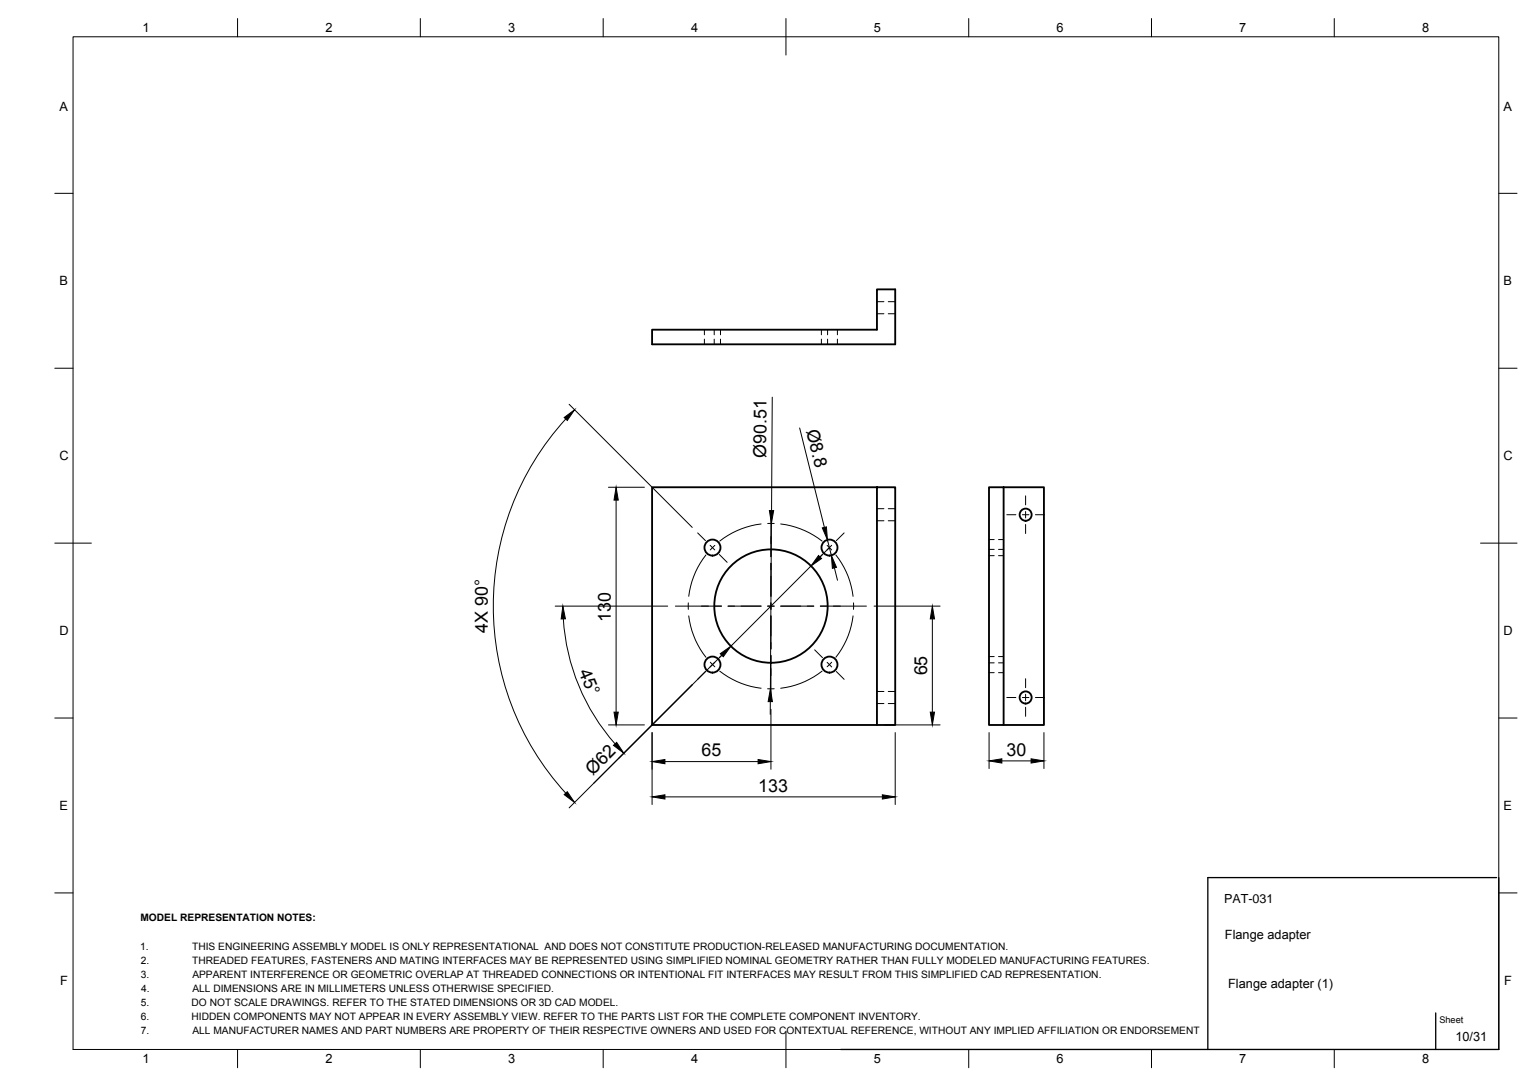
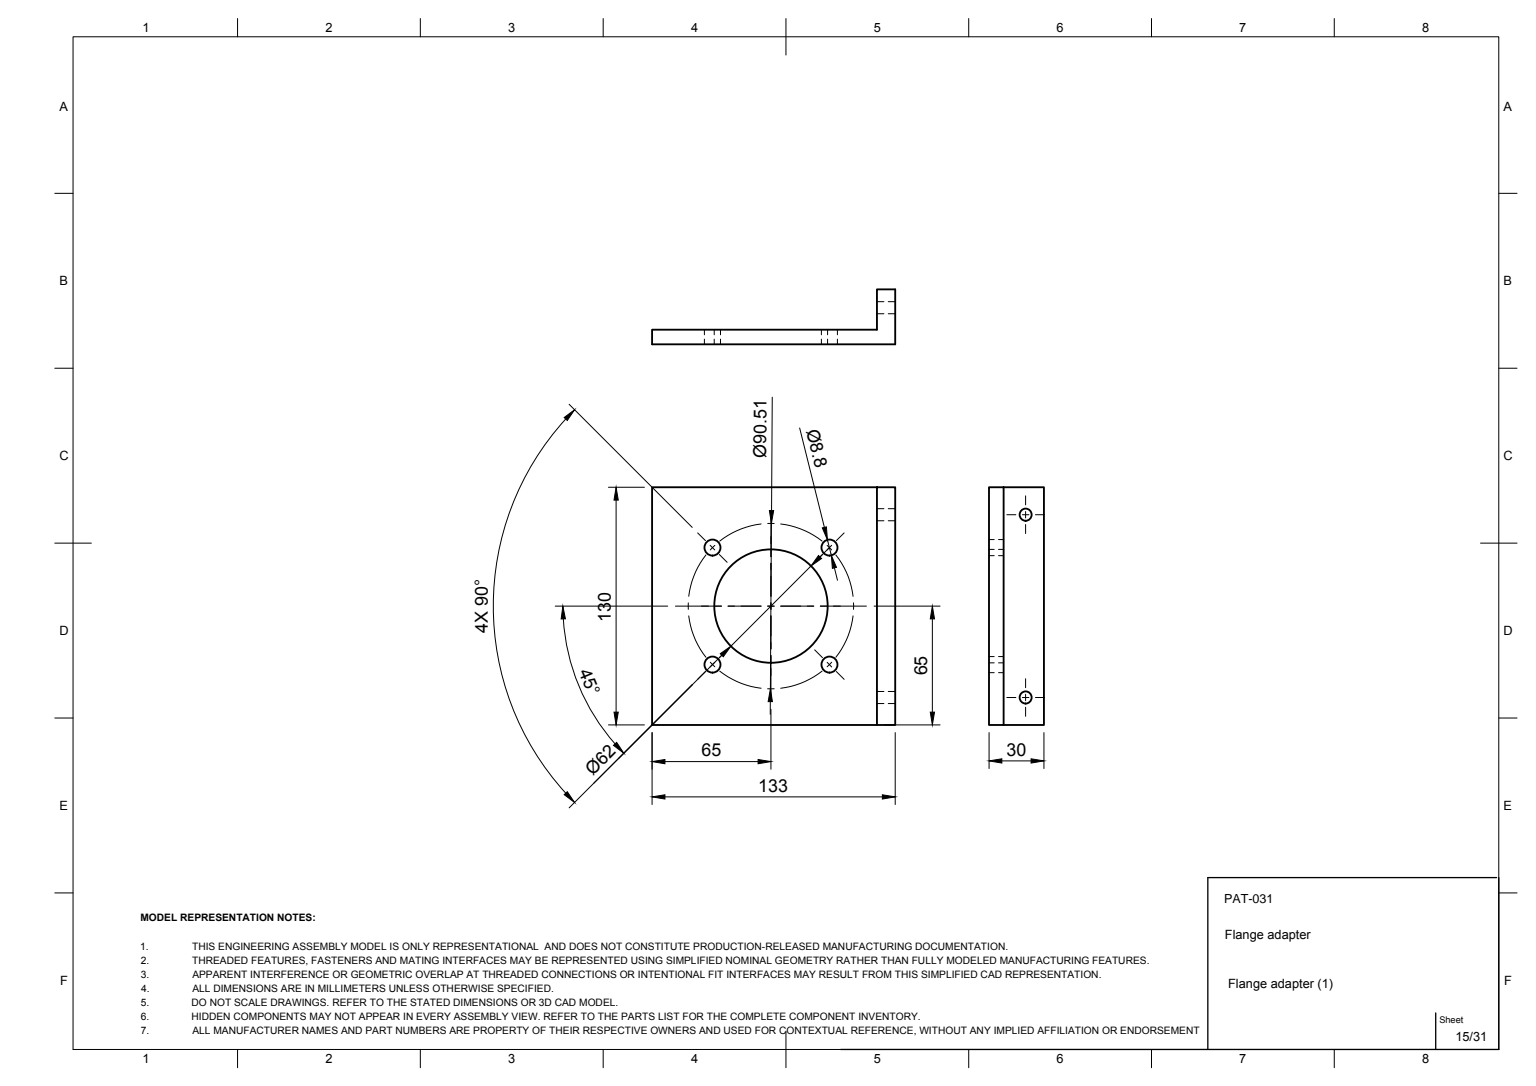
ISO-10303-21;
HEADER;
/* Generated by software containing ST-Developer
 * from STEP Tools, Inc. (www.steptools.com) 
 */

FILE_DESCRIPTION(
/* description */ ('Double-row support with tensioned shaft'),
/* implementation_level */ '2;1');

FILE_NAME(
/* name */ 'Flange adapter (1).step',
/* time_stamp */ '2026-10-27T10:50:35-07:00',
/* author */ (''),
/* organization */ (''),
/* preprocessor_version */ 'ST-DEVELOPER v20.2',
/* originating_system */ 'Autodesk Translation Framework v15.17.0.0',
/* authorisation */ '');

FILE_SCHEMA (('AUTOMOTIVE_DESIGN { 1 0 10303 214 3 1 1 }'));
ENDSEC;

DATA;
#10=MECHANICAL_DESIGN_GEOMETRIC_PRESENTATION_REPRESENTATION('',(#489),#11559);
#425=SHAPE_REPRESENTATION_RELATIONSHIP('SRR','None',#11733,#457);
#457=ADVANCED_BREP_SHAPE_REPRESENTATION('',(#522),#11535);
#489=STYLED_ITEM('',(#11953),#522);
#522=MANIFOLD_SOLID_BREP('Body1',#6334);
#588=FACE_BOUND('',#1388,.T.);
#589=FACE_BOUND('',#1389,.T.);
#590=FACE_BOUND('',#1392,.T.);
#591=FACE_BOUND('',#1393,.T.);
#592=FACE_BOUND('',#1394,.T.);
#593=FACE_BOUND('',#1395,.T.);
#594=FACE_BOUND('',#1396,.T.);
#595=FACE_BOUND('',#1400,.T.);
#596=FACE_BOUND('',#1401,.T.);
#597=FACE_BOUND('',#1402,.T.);
#598=FACE_BOUND('',#1403,.T.);
#599=FACE_BOUND('',#1404,.T.);
#600=FACE_BOUND('',#1407,.T.);
#601=FACE_BOUND('',#1408,.T.);
#725=PLANE('',#6874);
#726=PLANE('',#6875);
#727=PLANE('',#6876);
#728=PLANE('',#6877);
#729=PLANE('',#6878);
#730=PLANE('',#6879);
#731=PLANE('',#6880);
#732=PLANE('',#6881);
#990=FACE_OUTER_BOUND('',#1380,.T.);
#991=FACE_OUTER_BOUND('',#1381,.T.);
#992=FACE_OUTER_BOUND('',#1382,.T.);
#993=FACE_OUTER_BOUND('',#1383,.T.);
#994=FACE_OUTER_BOUND('',#1384,.T.);
#995=FACE_OUTER_BOUND('',#1385,.T.);
#996=FACE_OUTER_BOUND('',#1386,.T.);
#997=FACE_OUTER_BOUND('',#1387,.T.);
#998=FACE_OUTER_BOUND('',#1390,.T.);
#999=FACE_OUTER_BOUND('',#1391,.T.);
#1000=FACE_OUTER_BOUND('',#1397,.T.);
#1001=FACE_OUTER_BOUND('',#1398,.T.);
#1002=FACE_OUTER_BOUND('',#1399,.T.);
#1003=FACE_OUTER_BOUND('',#1405,.T.);
#1004=FACE_OUTER_BOUND('',#1406,.T.);
#1380=EDGE_LOOP('',(#4648,#4649,#4650,#4651));
#1381=EDGE_LOOP('',(#4652,#4653,#4654,#4655));
#1382=EDGE_LOOP('',(#4656,#4657,#4658,#4659));
#1383=EDGE_LOOP('',(#4660,#4661,#4662,#4663));
#1384=EDGE_LOOP('',(#4664,#4665,#4666,#4667));
#1385=EDGE_LOOP('',(#4668,#4669,#4670,#4671));
#1386=EDGE_LOOP('',(#4672,#4673,#4674,#4675));
#1387=EDGE_LOOP('',(#4676,#4677,#4678,#4679));
#1388=EDGE_LOOP('',(#4680));
#1389=EDGE_LOOP('',(#4681));
#1390=EDGE_LOOP('',(#4682,#4683,#4684,#4685));
#1391=EDGE_LOOP('',(#4686,#4687,#4688,#4689));
#1392=EDGE_LOOP('',(#4690));
#1393=EDGE_LOOP('',(#4691));
#1394=EDGE_LOOP('',(#4692));
#1395=EDGE_LOOP('',(#4693));
#1396=EDGE_LOOP('',(#4694));
#1397=EDGE_LOOP('',(#4695,#4696,#4697,#4698,#4699,#4700));
#1398=EDGE_LOOP('',(#4701,#4702,#4703,#4704,#4705,#4706));
#1399=EDGE_LOOP('',(#4707,#4708,#4709,#4710));
#1400=EDGE_LOOP('',(#4711));
#1401=EDGE_LOOP('',(#4712));
#1402=EDGE_LOOP('',(#4713));
#1403=EDGE_LOOP('',(#4714));
#1404=EDGE_LOOP('',(#4715));
#1405=EDGE_LOOP('',(#4716,#4717,#4718,#4719));
#1406=EDGE_LOOP('',(#4720,#4721,#4722,#4723));
#1407=EDGE_LOOP('',(#4724));
#1408=EDGE_LOOP('',(#4725));
#1847=LINE('',#9589,#2394);
#1848=LINE('',#9595,#2395);
#1849=LINE('',#9601,#2396);
#1850=LINE('',#9607,#2397);
#1851=LINE('',#9613,#2398);
#1852=LINE('',#9619,#2399);
#1853=LINE('',#9625,#2400);
#1854=LINE('',#9630,#2401);
#1855=LINE('',#9632,#2402);
#1856=LINE('',#9634,#2403);
#1857=LINE('',#9635,#2404);
#1858=LINE('',#9638,#2405);
#1859=LINE('',#9640,#2406);
#1860=LINE('',#9641,#2407);
#1861=LINE('',#9645,#2408);
#1862=LINE('',#9647,#2409);
#1863=LINE('',#9649,#2410);
#1864=LINE('',#9650,#2411);
#1865=LINE('',#9653,#2412);
#1866=LINE('',#9654,#2413);
#1867=LINE('',#9655,#2414);
#1868=LINE('',#9658,#2415);
#1869=LINE('',#9659,#2416);
#1870=LINE('',#9660,#2417);
#1871=LINE('',#9662,#2418);
#2394=VECTOR('',#7760,0.33);
#2395=VECTOR('',#7767,0.33);
#2396=VECTOR('',#7774,0.44);
#2397=VECTOR('',#7781,0.44);
#2398=VECTOR('',#7788,0.44);
#2399=VECTOR('',#7795,0.44);
#2400=VECTOR('',#7802,3.1);
#2401=VECTOR('',#7807,1.);
#2402=VECTOR('',#7808,1.);
#2403=VECTOR('',#7809,1.);
#2404=VECTOR('',#7810,1.);
#2405=VECTOR('',#7813,1.);
#2406=VECTOR('',#7814,1.);
#2407=VECTOR('',#7815,1.);
#2408=VECTOR('',#7818,1.);
#2409=VECTOR('',#7819,1.);
#2410=VECTOR('',#7820,1.);
#2411=VECTOR('',#7821,1.);
#2412=VECTOR('',#7824,1.);
#2413=VECTOR('',#7825,1.);
#2414=VECTOR('',#7826,1.);
#2415=VECTOR('',#7829,1.);
#2416=VECTOR('',#7830,1.);
#2417=VECTOR('',#7831,1.);
#2418=VECTOR('',#7834,1.);
#2890=CIRCLE('',#6854,0.33);
#2891=CIRCLE('',#6855,0.33);
#2892=CIRCLE('',#6857,0.33);
#2893=CIRCLE('',#6858,0.33);
#2894=CIRCLE('',#6860,0.44);
#2895=CIRCLE('',#6861,0.44);
#2896=CIRCLE('',#6863,0.44);
#2897=CIRCLE('',#6864,0.44);
#2898=CIRCLE('',#6866,0.44);
#2899=CIRCLE('',#6867,0.44);
#2900=CIRCLE('',#6869,0.44);
#2901=CIRCLE('',#6870,0.44);
#2902=CIRCLE('',#6872,3.1);
#2903=CIRCLE('',#6873,3.1);
#3133=VERTEX_POINT('',#9586);
#3134=VERTEX_POINT('',#9588);
#3135=VERTEX_POINT('',#9592);
#3136=VERTEX_POINT('',#9594);
#3137=VERTEX_POINT('',#9598);
#3138=VERTEX_POINT('',#9600);
#3139=VERTEX_POINT('',#9604);
#3140=VERTEX_POINT('',#9606);
#3141=VERTEX_POINT('',#9610);
#3142=VERTEX_POINT('',#9612);
#3143=VERTEX_POINT('',#9616);
#3144=VERTEX_POINT('',#9618);
#3145=VERTEX_POINT('',#9622);
#3146=VERTEX_POINT('',#9624);
#3147=VERTEX_POINT('',#9628);
#3148=VERTEX_POINT('',#9629);
#3149=VERTEX_POINT('',#9631);
#3150=VERTEX_POINT('',#9633);
#3151=VERTEX_POINT('',#9637);
#3152=VERTEX_POINT('',#9639);
#3153=VERTEX_POINT('',#9643);
#3154=VERTEX_POINT('',#9644);
#3155=VERTEX_POINT('',#9646);
#3156=VERTEX_POINT('',#9648);
#3157=VERTEX_POINT('',#9652);
#3158=VERTEX_POINT('',#9657);
#3709=EDGE_CURVE('',#3133,#3133,#2890,.T.);
#3710=EDGE_CURVE('',#3133,#3134,#1847,.T.);
#3711=EDGE_CURVE('',#3134,#3134,#2891,.T.);
#3712=EDGE_CURVE('',#3135,#3135,#2892,.T.);
#3713=EDGE_CURVE('',#3135,#3136,#1848,.T.);
#3714=EDGE_CURVE('',#3136,#3136,#2893,.T.);
#3715=EDGE_CURVE('',#3137,#3137,#2894,.T.);
#3716=EDGE_CURVE('',#3137,#3138,#1849,.T.);
#3717=EDGE_CURVE('',#3138,#3138,#2895,.T.);
#3718=EDGE_CURVE('',#3139,#3139,#2896,.T.);
#3719=EDGE_CURVE('',#3139,#3140,#1850,.T.);
#3720=EDGE_CURVE('',#3140,#3140,#2897,.T.);
#3721=EDGE_CURVE('',#3141,#3141,#2898,.T.);
#3722=EDGE_CURVE('',#3141,#3142,#1851,.T.);
#3723=EDGE_CURVE('',#3142,#3142,#2899,.T.);
#3724=EDGE_CURVE('',#3143,#3143,#2900,.T.);
#3725=EDGE_CURVE('',#3143,#3144,#1852,.T.);
#3726=EDGE_CURVE('',#3144,#3144,#2901,.T.);
#3727=EDGE_CURVE('',#3145,#3145,#2902,.T.);
#3728=EDGE_CURVE('',#3145,#3146,#1853,.T.);
#3729=EDGE_CURVE('',#3146,#3146,#2903,.T.);
#3730=EDGE_CURVE('',#3147,#3148,#1854,.T.);
#3731=EDGE_CURVE('',#3149,#3147,#1855,.T.);
#3732=EDGE_CURVE('',#3150,#3149,#1856,.T.);
#3733=EDGE_CURVE('',#3150,#3148,#1857,.T.);
#3734=EDGE_CURVE('',#3149,#3151,#1858,.T.);
#3735=EDGE_CURVE('',#3151,#3152,#1859,.T.);
#3736=EDGE_CURVE('',#3152,#3150,#1860,.T.);
#3737=EDGE_CURVE('',#3153,#3154,#1861,.T.);
#3738=EDGE_CURVE('',#3155,#3154,#1862,.T.);
#3739=EDGE_CURVE('',#3156,#3155,#1863,.T.);
#3740=EDGE_CURVE('',#3156,#3153,#1864,.T.);
#3741=EDGE_CURVE('',#3147,#3157,#1865,.T.);
#3742=EDGE_CURVE('',#3154,#3157,#1866,.T.);
#3743=EDGE_CURVE('',#3153,#3151,#1867,.T.);
#3744=EDGE_CURVE('',#3158,#3155,#1868,.T.);
#3745=EDGE_CURVE('',#3148,#3158,#1869,.T.);
#3746=EDGE_CURVE('',#3152,#3156,#1870,.T.);
#3747=EDGE_CURVE('',#3157,#3158,#1871,.T.);
#4648=ORIENTED_EDGE('',*,*,#3709,.F.);
#4649=ORIENTED_EDGE('',*,*,#3710,.T.);
#4650=ORIENTED_EDGE('',*,*,#3711,.F.);
#4651=ORIENTED_EDGE('',*,*,#3710,.F.);
#4652=ORIENTED_EDGE('',*,*,#3712,.F.);
#4653=ORIENTED_EDGE('',*,*,#3713,.T.);
#4654=ORIENTED_EDGE('',*,*,#3714,.F.);
#4655=ORIENTED_EDGE('',*,*,#3713,.F.);
#4656=ORIENTED_EDGE('',*,*,#3715,.F.);
#4657=ORIENTED_EDGE('',*,*,#3716,.T.);
#4658=ORIENTED_EDGE('',*,*,#3717,.F.);
#4659=ORIENTED_EDGE('',*,*,#3716,.F.);
#4660=ORIENTED_EDGE('',*,*,#3718,.F.);
#4661=ORIENTED_EDGE('',*,*,#3719,.T.);
#4662=ORIENTED_EDGE('',*,*,#3720,.F.);
#4663=ORIENTED_EDGE('',*,*,#3719,.F.);
#4664=ORIENTED_EDGE('',*,*,#3721,.F.);
#4665=ORIENTED_EDGE('',*,*,#3722,.T.);
#4666=ORIENTED_EDGE('',*,*,#3723,.F.);
#4667=ORIENTED_EDGE('',*,*,#3722,.F.);
#4668=ORIENTED_EDGE('',*,*,#3724,.F.);
#4669=ORIENTED_EDGE('',*,*,#3725,.T.);
#4670=ORIENTED_EDGE('',*,*,#3726,.F.);
#4671=ORIENTED_EDGE('',*,*,#3725,.F.);
#4672=ORIENTED_EDGE('',*,*,#3727,.F.);
#4673=ORIENTED_EDGE('',*,*,#3728,.T.);
#4674=ORIENTED_EDGE('',*,*,#3729,.F.);
#4675=ORIENTED_EDGE('',*,*,#3728,.F.);
#4676=ORIENTED_EDGE('',*,*,#3730,.F.);
#4677=ORIENTED_EDGE('',*,*,#3731,.F.);
#4678=ORIENTED_EDGE('',*,*,#3732,.F.);
#4679=ORIENTED_EDGE('',*,*,#3733,.T.);
#4680=ORIENTED_EDGE('',*,*,#3711,.T.);
#4681=ORIENTED_EDGE('',*,*,#3714,.T.);
#4682=ORIENTED_EDGE('',*,*,#3732,.T.);
#4683=ORIENTED_EDGE('',*,*,#3734,.T.);
#4684=ORIENTED_EDGE('',*,*,#3735,.T.);
#4685=ORIENTED_EDGE('',*,*,#3736,.T.);
#4686=ORIENTED_EDGE('',*,*,#3737,.T.);
#4687=ORIENTED_EDGE('',*,*,#3738,.F.);
#4688=ORIENTED_EDGE('',*,*,#3739,.F.);
#4689=ORIENTED_EDGE('',*,*,#3740,.T.);
#4690=ORIENTED_EDGE('',*,*,#3729,.T.);
#4691=ORIENTED_EDGE('',*,*,#3726,.T.);
#4692=ORIENTED_EDGE('',*,*,#3723,.T.);
#4693=ORIENTED_EDGE('',*,*,#3720,.T.);
#4694=ORIENTED_EDGE('',*,*,#3717,.T.);
#4695=ORIENTED_EDGE('',*,*,#3741,.T.);
#4696=ORIENTED_EDGE('',*,*,#3742,.F.);
#4697=ORIENTED_EDGE('',*,*,#3737,.F.);
#4698=ORIENTED_EDGE('',*,*,#3743,.T.);
#4699=ORIENTED_EDGE('',*,*,#3734,.F.);
#4700=ORIENTED_EDGE('',*,*,#3731,.T.);
#4701=ORIENTED_EDGE('',*,*,#3739,.T.);
#4702=ORIENTED_EDGE('',*,*,#3744,.F.);
#4703=ORIENTED_EDGE('',*,*,#3745,.F.);
#4704=ORIENTED_EDGE('',*,*,#3733,.F.);
#4705=ORIENTED_EDGE('',*,*,#3736,.F.);
#4706=ORIENTED_EDGE('',*,*,#3746,.T.);
#4707=ORIENTED_EDGE('',*,*,#3730,.T.);
#4708=ORIENTED_EDGE('',*,*,#3745,.T.);
#4709=ORIENTED_EDGE('',*,*,#3747,.F.);
#4710=ORIENTED_EDGE('',*,*,#3741,.F.);
#4711=ORIENTED_EDGE('',*,*,#3727,.T.);
#4712=ORIENTED_EDGE('',*,*,#3724,.T.);
#4713=ORIENTED_EDGE('',*,*,#3721,.T.);
#4714=ORIENTED_EDGE('',*,*,#3718,.T.);
#4715=ORIENTED_EDGE('',*,*,#3715,.T.);
#4716=ORIENTED_EDGE('',*,*,#3742,.T.);
#4717=ORIENTED_EDGE('',*,*,#3747,.T.);
#4718=ORIENTED_EDGE('',*,*,#3744,.T.);
#4719=ORIENTED_EDGE('',*,*,#3738,.T.);
#4720=ORIENTED_EDGE('',*,*,#3743,.F.);
#4721=ORIENTED_EDGE('',*,*,#3740,.F.);
#4722=ORIENTED_EDGE('',*,*,#3746,.F.);
#4723=ORIENTED_EDGE('',*,*,#3735,.F.);
#4724=ORIENTED_EDGE('',*,*,#3709,.T.);
#4725=ORIENTED_EDGE('',*,*,#3712,.T.);
#5917=CYLINDRICAL_SURFACE('',#6853,0.33);
#5918=CYLINDRICAL_SURFACE('',#6856,0.33);
#5919=CYLINDRICAL_SURFACE('',#6859,0.44);
#5920=CYLINDRICAL_SURFACE('',#6862,0.44);
#5921=CYLINDRICAL_SURFACE('',#6865,0.44);
#5922=CYLINDRICAL_SURFACE('',#6868,0.44);
#5923=CYLINDRICAL_SURFACE('',#6871,3.1);
#6053=ADVANCED_FACE('',(#990),#5917,.F.);
#6054=ADVANCED_FACE('',(#991),#5918,.F.);
#6055=ADVANCED_FACE('',(#992),#5919,.F.);
#6056=ADVANCED_FACE('',(#993),#5920,.F.);
#6057=ADVANCED_FACE('',(#994),#5921,.F.);
#6058=ADVANCED_FACE('',(#995),#5922,.F.);
#6059=ADVANCED_FACE('',(#996),#5923,.F.);
#6060=ADVANCED_FACE('',(#997,#588,#589),#725,.T.);
#6061=ADVANCED_FACE('',(#998),#726,.F.);
#6062=ADVANCED_FACE('',(#999,#590,#591,#592,#593,#594),#727,.T.);
#6063=ADVANCED_FACE('',(#1000),#728,.T.);
#6064=ADVANCED_FACE('',(#1001),#729,.T.);
#6065=ADVANCED_FACE('',(#1002,#595,#596,#597,#598,#599),#730,.T.);
#6066=ADVANCED_FACE('',(#1003),#731,.T.);
#6067=ADVANCED_FACE('',(#1004,#600,#601),#732,.F.);
#6334=CLOSED_SHELL('',(#6053,#6054,#6055,#6056,#6057,#6058,#6059,#6060,
#6061,#6062,#6063,#6064,#6065,#6066,#6067));
#6852=AXIS2_PLACEMENT_3D('',#9584,#7754,#7755);
#6853=AXIS2_PLACEMENT_3D('',#9585,#7756,#7757);
#6854=AXIS2_PLACEMENT_3D('',#9587,#7758,#7759);
#6855=AXIS2_PLACEMENT_3D('',#9590,#7761,#7762);
#6856=AXIS2_PLACEMENT_3D('',#9591,#7763,#7764);
#6857=AXIS2_PLACEMENT_3D('',#9593,#7765,#7766);
#6858=AXIS2_PLACEMENT_3D('',#9596,#7768,#7769);
#6859=AXIS2_PLACEMENT_3D('',#9597,#7770,#7771);
#6860=AXIS2_PLACEMENT_3D('',#9599,#7772,#7773);
#6861=AXIS2_PLACEMENT_3D('',#9602,#7775,#7776);
#6862=AXIS2_PLACEMENT_3D('',#9603,#7777,#7778);
#6863=AXIS2_PLACEMENT_3D('',#9605,#7779,#7780);
#6864=AXIS2_PLACEMENT_3D('',#9608,#7782,#7783);
#6865=AXIS2_PLACEMENT_3D('',#9609,#7784,#7785);
#6866=AXIS2_PLACEMENT_3D('',#9611,#7786,#7787);
#6867=AXIS2_PLACEMENT_3D('',#9614,#7789,#7790);
#6868=AXIS2_PLACEMENT_3D('',#9615,#7791,#7792);
#6869=AXIS2_PLACEMENT_3D('',#9617,#7793,#7794);
#6870=AXIS2_PLACEMENT_3D('',#9620,#7796,#7797);
#6871=AXIS2_PLACEMENT_3D('',#9621,#7798,#7799);
#6872=AXIS2_PLACEMENT_3D('',#9623,#7800,#7801);
#6873=AXIS2_PLACEMENT_3D('',#9626,#7803,#7804);
#6874=AXIS2_PLACEMENT_3D('',#9627,#7805,#7806);
#6875=AXIS2_PLACEMENT_3D('',#9636,#7811,#7812);
#6876=AXIS2_PLACEMENT_3D('',#9642,#7816,#7817);
#6877=AXIS2_PLACEMENT_3D('',#9651,#7822,#7823);
#6878=AXIS2_PLACEMENT_3D('',#9656,#7827,#7828);
#6879=AXIS2_PLACEMENT_3D('',#9661,#7832,#7833);
#6880=AXIS2_PLACEMENT_3D('',#9663,#7835,#7836);
#6881=AXIS2_PLACEMENT_3D('',#9664,#7837,#7838);
#7754=DIRECTION('axis',(0.,0.,1.));
#7755=DIRECTION('refdir',(1.,0.,0.));
#7756=DIRECTION('center_axis',(0.,0.,1.));
#7757=DIRECTION('ref_axis',(1.,0.,0.));
#7758=DIRECTION('center_axis',(0.,0.,1.));
#7759=DIRECTION('ref_axis',(1.,0.,0.));
#7760=DIRECTION('',(0.,0.,1.));
#7761=DIRECTION('center_axis',(0.,0.,-1.));
#7762=DIRECTION('ref_axis',(1.,0.,0.));
#7763=DIRECTION('center_axis',(0.,0.,1.));
#7764=DIRECTION('ref_axis',(1.,0.,0.));
#7765=DIRECTION('center_axis',(0.,0.,1.));
#7766=DIRECTION('ref_axis',(1.,0.,0.));
#7767=DIRECTION('',(0.,0.,1.));
#7768=DIRECTION('center_axis',(0.,0.,-1.));
#7769=DIRECTION('ref_axis',(1.,0.,0.));
#7770=DIRECTION('center_axis',(0.,1.,0.));
#7771=DIRECTION('ref_axis',(1.,0.,0.));
#7772=DIRECTION('center_axis',(0.,1.,0.));
#7773=DIRECTION('ref_axis',(1.,0.,0.));
#7774=DIRECTION('',(0.,1.,0.));
#7775=DIRECTION('center_axis',(0.,-1.,0.));
#7776=DIRECTION('ref_axis',(1.,0.,0.));
#7777=DIRECTION('center_axis',(0.,1.,0.));
#7778=DIRECTION('ref_axis',(1.,0.,0.));
#7779=DIRECTION('center_axis',(0.,1.,0.));
#7780=DIRECTION('ref_axis',(1.,0.,0.));
#7781=DIRECTION('',(0.,1.,0.));
#7782=DIRECTION('center_axis',(0.,-1.,0.));
#7783=DIRECTION('ref_axis',(1.,0.,0.));
#7784=DIRECTION('center_axis',(0.,1.,0.));
#7785=DIRECTION('ref_axis',(1.,0.,0.));
#7786=DIRECTION('center_axis',(0.,1.,0.));
#7787=DIRECTION('ref_axis',(1.,0.,0.));
#7788=DIRECTION('',(0.,1.,0.));
#7789=DIRECTION('center_axis',(0.,-1.,0.));
#7790=DIRECTION('ref_axis',(1.,0.,0.));
#7791=DIRECTION('center_axis',(0.,1.,0.));
#7792=DIRECTION('ref_axis',(1.,0.,0.));
#7793=DIRECTION('center_axis',(0.,1.,0.));
#7794=DIRECTION('ref_axis',(1.,0.,0.));
#7795=DIRECTION('',(0.,1.,0.));
#7796=DIRECTION('center_axis',(0.,-1.,0.));
#7797=DIRECTION('ref_axis',(1.,0.,0.));
#7798=DIRECTION('center_axis',(0.,1.,0.));
#7799=DIRECTION('ref_axis',(1.,0.,0.));
#7800=DIRECTION('center_axis',(0.,1.,0.));
#7801=DIRECTION('ref_axis',(1.,0.,0.));
#7802=DIRECTION('',(0.,1.,0.));
#7803=DIRECTION('center_axis',(0.,-1.,0.));
#7804=DIRECTION('ref_axis',(1.,0.,0.));
#7805=DIRECTION('center_axis',(0.,0.,1.));
#7806=DIRECTION('ref_axis',(1.,0.,0.));
#7807=DIRECTION('',(1.,0.,0.));
#7808=DIRECTION('',(0.,1.,0.));
#7809=DIRECTION('',(-1.,0.,0.));
#7810=DIRECTION('',(0.,1.,0.));
#7811=DIRECTION('center_axis',(0.,1.,0.));
#7812=DIRECTION('ref_axis',(1.,0.,0.));
#7813=DIRECTION('',(0.,0.,-1.));
#7814=DIRECTION('',(1.,0.,0.));
#7815=DIRECTION('',(0.,0.,1.));
#7816=DIRECTION('center_axis',(0.,1.,0.));
#7817=DIRECTION('ref_axis',(-1.,0.,0.));
#7818=DIRECTION('',(0.,0.,1.));
#7819=DIRECTION('',(-1.,0.,0.));
#7820=DIRECTION('',(0.,0.,1.));
#7821=DIRECTION('',(-1.,0.,0.));
#7822=DIRECTION('center_axis',(-1.,0.,0.));
#7823=DIRECTION('ref_axis',(0.,-1.,0.));
#7824=DIRECTION('',(0.,0.,1.));
#7825=DIRECTION('',(0.,-1.,0.));
#7826=DIRECTION('',(0.,-1.,0.));
#7827=DIRECTION('center_axis',(1.,0.,0.));
#7828=DIRECTION('ref_axis',(0.,1.,0.));
#7829=DIRECTION('',(0.,1.,0.));
#7830=DIRECTION('',(0.,0.,1.));
#7831=DIRECTION('',(0.,1.,0.));
#7832=DIRECTION('center_axis',(0.,-1.,0.));
#7833=DIRECTION('ref_axis',(1.,0.,0.));
#7834=DIRECTION('',(1.,0.,0.));
#7835=DIRECTION('center_axis',(0.,0.,1.));
#7836=DIRECTION('ref_axis',(1.,0.,0.));
#7837=DIRECTION('center_axis',(0.,0.,1.));
#7838=DIRECTION('ref_axis',(1.,0.,0.));
#9584=CARTESIAN_POINT('',(0.,0.,0.));
#9585=CARTESIAN_POINT('Origin',(-5.,15.5,3.1));
#9586=CARTESIAN_POINT('',(-5.33,15.5,3.2));
#9587=CARTESIAN_POINT('Origin',(-5.,15.5,3.2));
#9588=CARTESIAN_POINT('',(-5.33,15.5,4.2));
#9589=CARTESIAN_POINT('',(-5.33,15.5,3.1));
#9590=CARTESIAN_POINT('Origin',(-5.,15.5,4.2));
#9591=CARTESIAN_POINT('Origin',(5.,15.5,3.1));
#9592=CARTESIAN_POINT('',(4.67,15.5,3.2));
#9593=CARTESIAN_POINT('Origin',(5.,15.5,3.2));
#9594=CARTESIAN_POINT('',(4.67,15.5,4.2));
#9595=CARTESIAN_POINT('',(4.67,15.5,3.1));
#9596=CARTESIAN_POINT('Origin',(5.,15.5,4.2));
#9597=CARTESIAN_POINT('Origin',(3.2,16.6,6.8));
#9598=CARTESIAN_POINT('',(2.76,16.7,6.8));
#9599=CARTESIAN_POINT('Origin',(3.2,16.7,6.8));
#9600=CARTESIAN_POINT('',(2.76,17.5,6.8));
#9601=CARTESIAN_POINT('',(2.76,16.6,6.8));
#9602=CARTESIAN_POINT('Origin',(3.2,17.5,6.8));
#9603=CARTESIAN_POINT('Origin',(-3.2,16.6,13.2));
#9604=CARTESIAN_POINT('',(-3.64,16.7,13.2));
#9605=CARTESIAN_POINT('Origin',(-3.2,16.7,13.2));
#9606=CARTESIAN_POINT('',(-3.64,17.5,13.2));
#9607=CARTESIAN_POINT('',(-3.64,16.6,13.2));
#9608=CARTESIAN_POINT('Origin',(-3.2,17.5,13.2));
#9609=CARTESIAN_POINT('Origin',(-3.2,16.6,6.8));
#9610=CARTESIAN_POINT('',(-3.64,16.7,6.8));
#9611=CARTESIAN_POINT('Origin',(-3.2,16.7,6.8));
#9612=CARTESIAN_POINT('',(-3.64,17.5,6.8));
#9613=CARTESIAN_POINT('',(-3.64,16.6,6.8));
#9614=CARTESIAN_POINT('Origin',(-3.2,17.5,6.8));
#9615=CARTESIAN_POINT('Origin',(3.2,16.6,13.2));
#9616=CARTESIAN_POINT('',(2.76,16.7,13.2));
#9617=CARTESIAN_POINT('Origin',(3.2,16.7,13.2));
#9618=CARTESIAN_POINT('',(2.76,17.5,13.2));
#9619=CARTESIAN_POINT('',(2.76,16.6,13.2));
#9620=CARTESIAN_POINT('Origin',(3.2,17.5,13.2));
#9621=CARTESIAN_POINT('Origin',(0.,16.6,10.));
#9622=CARTESIAN_POINT('',(-3.1,16.7,10.));
#9623=CARTESIAN_POINT('Origin',(0.,16.7,10.));
#9624=CARTESIAN_POINT('',(-3.1,17.5,10.));
#9625=CARTESIAN_POINT('',(-3.1,16.6,10.));
#9626=CARTESIAN_POINT('Origin',(0.,17.5,10.));
#9627=CARTESIAN_POINT('Origin',(-6.5,14.5,4.2));
#9628=CARTESIAN_POINT('',(-6.5,16.7,4.2));
#9629=CARTESIAN_POINT('',(6.5,16.7,4.2));
#9630=CARTESIAN_POINT('',(-6.5,16.7,4.2));
#9631=CARTESIAN_POINT('',(-6.5,14.5,4.2));
#9632=CARTESIAN_POINT('',(-6.5,14.5,4.2));
#9633=CARTESIAN_POINT('',(6.5,14.5,4.2));
#9634=CARTESIAN_POINT('',(6.5,14.5,4.2));
#9635=CARTESIAN_POINT('',(6.5,14.5,4.2));
#9636=CARTESIAN_POINT('Origin',(0.,14.5,3.7));
#9637=CARTESIAN_POINT('',(-6.5,14.5,3.2));
#9638=CARTESIAN_POINT('',(-6.5,14.5,4.2));
#9639=CARTESIAN_POINT('',(6.5,14.5,3.2));
#9640=CARTESIAN_POINT('',(-6.5,14.5,3.2));
#9641=CARTESIAN_POINT('',(6.5,14.5,3.2));
#9642=CARTESIAN_POINT('Origin',(6.5,17.5,3.2));
#9643=CARTESIAN_POINT('',(-6.5,17.5,3.2));
#9644=CARTESIAN_POINT('',(-6.5,17.5,16.5));
#9645=CARTESIAN_POINT('',(-6.5,17.5,3.2));
#9646=CARTESIAN_POINT('',(6.5,17.5,16.5));
#9647=CARTESIAN_POINT('',(6.5,17.5,16.5));
#9648=CARTESIAN_POINT('',(6.5,17.5,3.2));
#9649=CARTESIAN_POINT('',(6.5,17.5,3.2));
#9650=CARTESIAN_POINT('',(6.5,17.5,3.2));
#9651=CARTESIAN_POINT('Origin',(-6.5,17.5,3.2));
#9652=CARTESIAN_POINT('',(-6.5,16.7,16.5));
#9653=CARTESIAN_POINT('',(-6.5,16.7,3.2));
#9654=CARTESIAN_POINT('',(-6.5,17.5,16.5));
#9655=CARTESIAN_POINT('',(-6.5,17.5,3.2));
#9656=CARTESIAN_POINT('Origin',(6.5,16.7,3.2));
#9657=CARTESIAN_POINT('',(6.5,16.7,16.5));
#9658=CARTESIAN_POINT('',(6.5,16.7,16.5));
#9659=CARTESIAN_POINT('',(6.5,16.7,3.2));
#9660=CARTESIAN_POINT('',(6.5,14.5,3.2));
#9661=CARTESIAN_POINT('Origin',(-6.5,16.7,3.2));
#9662=CARTESIAN_POINT('',(-6.5,16.7,16.5));
#9663=CARTESIAN_POINT('Origin',(0.,17.1,16.5));
#9664=CARTESIAN_POINT('Origin',(0.,17.1,3.2));
#11498=UNCERTAINTY_MEASURE_WITH_UNIT(LENGTH_MEASURE(0.001),#11560,
'DISTANCE_ACCURACY_VALUE',
'Maximum model space distance between geometric entities at asserted c
onnectivities');
#11522=UNCERTAINTY_MEASURE_WITH_UNIT(LENGTH_MEASURE(0.001),#11560,
'DISTANCE_ACCURACY_VALUE',
'Maximum model space distance between geometric entities at asserted c
onnectivities');
#11535=(
GEOMETRIC_REPRESENTATION_CONTEXT(3)
GLOBAL_UNCERTAINTY_ASSIGNED_CONTEXT((#11498))
GLOBAL_UNIT_ASSIGNED_CONTEXT((#11560,#11562,#11563))
REPRESENTATION_CONTEXT('','3D')
);
#11559=(
GEOMETRIC_REPRESENTATION_CONTEXT(3)
GLOBAL_UNCERTAINTY_ASSIGNED_CONTEXT((#11522))
GLOBAL_UNIT_ASSIGNED_CONTEXT((#11560,#11562,#11563))
REPRESENTATION_CONTEXT('','3D')
);
#11560=(
LENGTH_UNIT()
NAMED_UNIT(*)
SI_UNIT(.CENTI.,.METRE.)
);
#11562=(
NAMED_UNIT(*)
PLANE_ANGLE_UNIT()
SI_UNIT($,.RADIAN.)
);
#11563=(
NAMED_UNIT(*)
SI_UNIT($,.STERADIAN.)
SOLID_ANGLE_UNIT()
);
#11576=SHAPE_DEFINITION_REPRESENTATION(#11612,#11733);
#11612=PRODUCT_DEFINITION_SHAPE('',$,#11770);
#11733=SHAPE_REPRESENTATION('',(#6852),#11535);
#11757=PRODUCT_DEFINITION_CONTEXT('part definition',#11867,'design');
#11770=PRODUCT_DEFINITION('Flange adapter (1)','Flange adapter (1)',#11806,
#11757);
#11806=PRODUCT_DEFINITION_FORMATION('',$,#11881);
#11867=APPLICATION_CONTEXT(
'Core Data for Automotive Mechanical Design Process');
#11868=PRODUCT_CONTEXT('part definition',#11867,'mechanical');
#11881=PRODUCT('Flange adapter (1)','Flange adapter (1)','Flange adapter (1)',
(#11868));
#11947=COLOUR_RGB('Light Blue',0.38,0.62,0.78);
#11948=FILL_AREA_STYLE_COLOUR('',#11947);
#11949=FILL_AREA_STYLE('',(#11948));
#11950=SURFACE_STYLE_FILL_AREA(#11949);
#11951=SURFACE_SIDE_STYLE('',(#11950));
#11952=SURFACE_STYLE_USAGE(.BOTH.,#11951);
#11953=PRESENTATION_STYLE_ASSIGNMENT((#11952));
ENDSEC;
END-ISO-10303-21;
